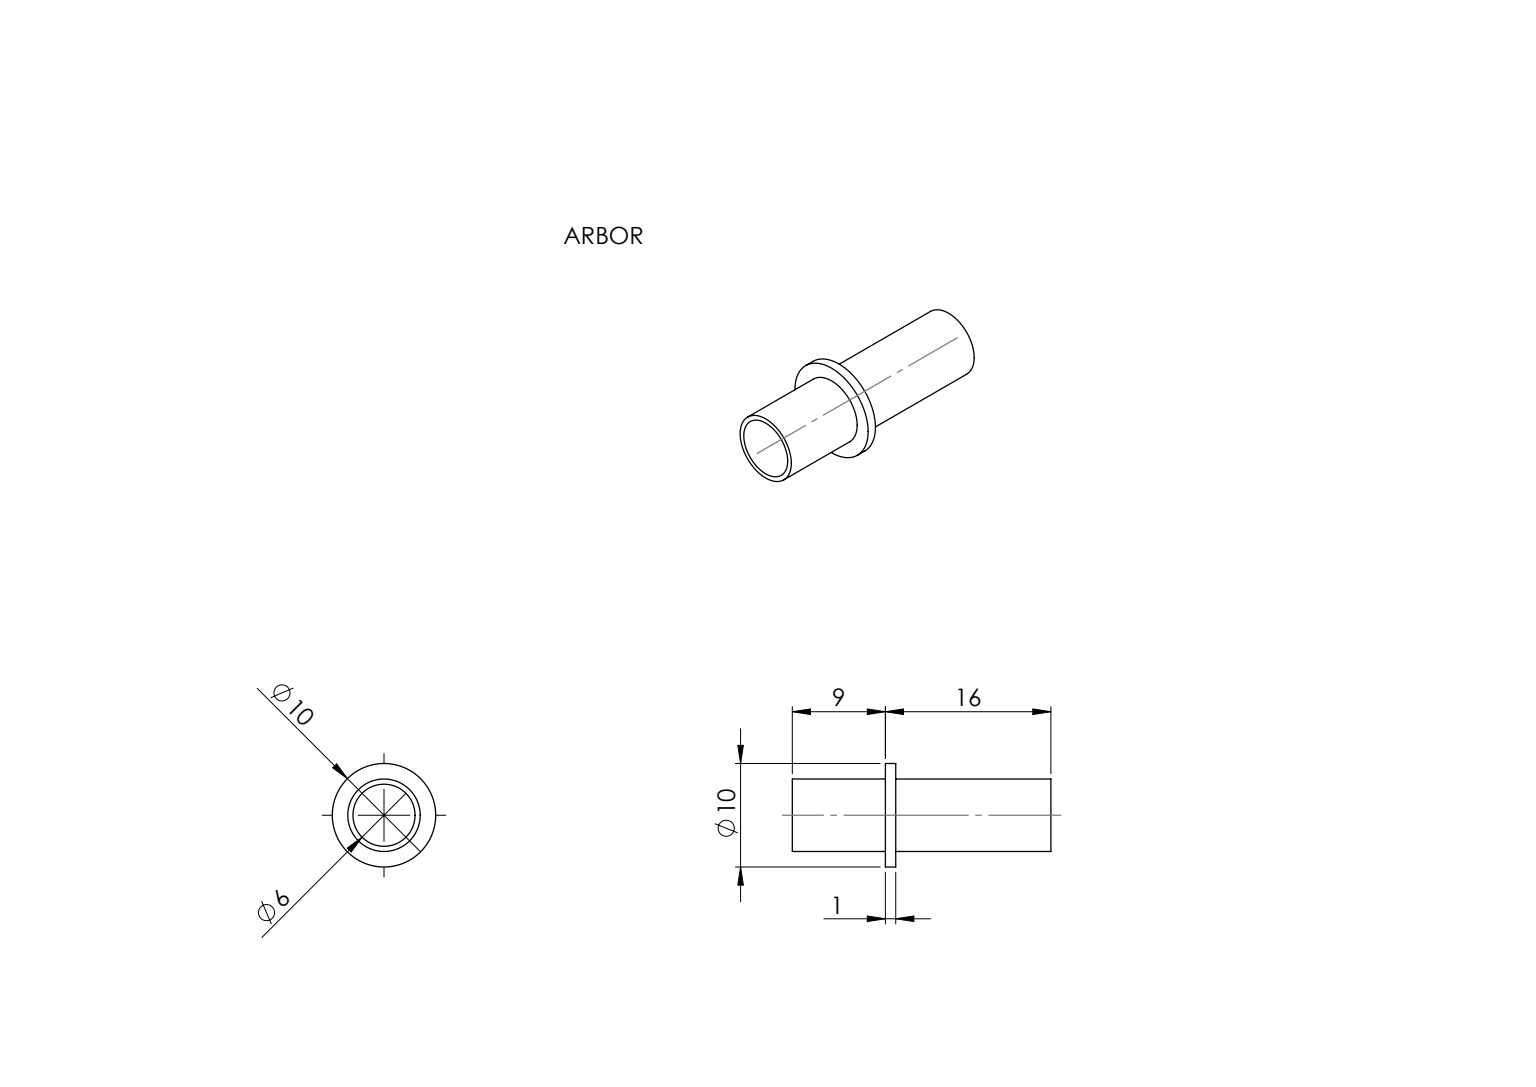
ISO-10303-21;
HEADER;
FILE_DESCRIPTION (('STEP AP214'),
    '1' );
FILE_NAME ('arbor.step',
    '2026-10-08T12:30:53',
    ( '' ),
    ( '' ),
    'SwSTEP 2.0',
    'SolidWorks 2026',
    '' );
FILE_SCHEMA (( 'AUTOMOTIVE_DESIGN' ));
ENDSEC;

DATA;
#87=DIRECTION ( 'NONE',  ( 1.000000000000000000, 0.000000000000000000, 0.000000000000000000 ) ) ;
#239=ORIENTED_EDGE ( 'NONE', *, *, #8409, .T. ) ;
#250=EDGE_LOOP ( 'NONE', ( #5066, #8144, #4716, #4779 ) ) ;
#253=AXIS2_PLACEMENT_3D ( 'NONE', #6645, #1940, #12036 ) ;
#365=EDGE_LOOP ( 'NONE', ( #9600, #8679, #4955, #8031 ) ) ;
#375=DIRECTION ( 'NONE',  ( 0.000000000000000000, 0.000000000000000000, 1.000000000000000000 ) ) ;
#462=EDGE_CURVE ( 'NONE', #4079, #6675, #6924, .T. ) ;
#471=EDGE_LOOP ( 'NONE', ( #5188, #8628, #9006, #4978 ) ) ;
#479=CARTESIAN_POINT ( 'NONE',  ( 0.000000000000000000, 0.000000000000000000, -15.00000000000000000 ) ) ;
#483=MANIFOLD_SOLID_BREP ( 'Boss-Extrude1', #814 ) ;
#506=DIRECTION ( 'NONE',  ( 0.000000000000000000, 0.000000000000000000, 1.000000000000000000 ) ) ;
#541=CARTESIAN_POINT ( 'NONE',  ( 0.000000000000000000, 0.000000000000000000, 1.000000000000000000 ) ) ;
#546=EDGE_LOOP ( 'NONE', ( #8097, #7998 ) ) ;
#571=DIRECTION ( 'NONE',  ( 0.000000000000000000, 0.000000000000000000, 1.000000000000000000 ) ) ;
#619=EDGE_CURVE ( 'NONE', #6675, #1739, #4934, .T. ) ;
#642=LINE ( 'NONE', #3336, #1232 ) ;
#668=FACE_OUTER_BOUND ( 'NONE', #4480, .T. ) ;
#682=EDGE_CURVE ( 'NONE', #9917, #762, #11766, .T. ) ;
#752=( LENGTH_UNIT ( ) NAMED_UNIT ( * ) SI_UNIT ( .MILLI., .METRE. ) );
#762=VERTEX_POINT ( 'NONE', #5708 ) ;
#781=FACE_OUTER_BOUND ( 'NONE', #365, .T. ) ;
#783=DIRECTION ( 'NONE',  ( -0.000000000000000000, -0.000000000000000000, -1.000000000000000000 ) ) ;
#814=CLOSED_SHELL ( 'NONE', ( #10354, #9816, #7402, #7243, #7988, #5762, #1031, #7711, #7647, #5316, #9141, #9675 ) ) ;
#820=DIRECTION ( 'NONE',  ( 1.000000000000000000, 0.000000000000000000, 0.000000000000000000 ) ) ;
#843=VERTEX_POINT ( 'NONE', #1693 ) ;
#927=SURFACE_SIDE_STYLE ('',( #10231 ) ) ;
#967=FACE_BOUND ( 'NONE', #8620, .T. ) ;
#972=AXIS2_PLACEMENT_3D ( 'NONE', #7512, #3791, #8558 ) ;
#1020=CARTESIAN_POINT ( 'NONE',  ( 0.000000000000000000, 0.000000000000000000, 0.000000000000000000 ) ) ;
#1031=ADVANCED_FACE ( 'NONE', ( #3715, #5556 ), #2860, .F. ) ;
#1041=CIRCLE ( 'NONE', #3776, 5.000000000000000000 ) ;
#1061=EDGE_CURVE ( 'NONE', #1959, #9571, #11360, .T. ) ;
#1065=( LENGTH_UNIT ( ) NAMED_UNIT ( * ) SI_UNIT ( .MILLI., .METRE. ) );
#1078=CARTESIAN_POINT ( 'NONE',  ( 0.000000000000000000, 0.000000000000000000, 0.000000000000000000 ) ) ;
#1088=FACE_OUTER_BOUND ( 'NONE', #9309, .T. ) ;
#1202=AXIS2_PLACEMENT_3D ( 'NONE', #1748, #5741, #6528 ) ;
#1232=VECTOR ( 'NONE', #6392, 1000.000000000000000 ) ;
#1264=CARTESIAN_POINT ( 'NONE',  ( 0.000000000000000000, 0.000000000000000000, 0.000000000000000000 ) ) ;
#1298=CYLINDRICAL_SURFACE ( 'NONE', #1709, 3.000000000000000000 ) ;
#1299=CARTESIAN_POINT ( 'NONE',  ( 0.000000000000000000, 0.000000000000000000, 10.00000000000000000 ) ) ;
#1301=EDGE_CURVE ( 'NONE', #3060, #5151, #1371, .T. ) ;
#1326=ADVANCED_BREP_SHAPE_REPRESENTATION ( '', ( #483, #8474 ), #1578 ) ;
#1371=CIRCLE ( 'NONE', #6829, 5.000000000000000000 ) ;
#1374=DIRECTION ( 'NONE',  ( 1.000000000000000000, 0.000000000000000000, 0.000000000000000000 ) ) ;
#1389=EDGE_CURVE ( 'NONE', #843, #3060, #7055, .T. ) ;
#1433=DIRECTION ( 'NONE',  ( 1.000000000000000000, 0.000000000000000000, 0.000000000000000000 ) ) ;
#1476=CIRCLE ( 'NONE', #5971, 3.500000000000000000 ) ;
#1493=DIRECTION ( 'NONE',  ( 1.000000000000000000, 0.000000000000000000, -0.000000000000000000 ) ) ;
#1551=DIRECTION ( 'NONE',  ( 0.000000000000000000, 0.000000000000000000, 1.000000000000000000 ) ) ;
#1578=( GEOMETRIC_REPRESENTATION_CONTEXT ( 3 ) GLOBAL_UNCERTAINTY_ASSIGNED_CONTEXT ( ( #2564 ) ) GLOBAL_UNIT_ASSIGNED_CONTEXT ( ( #752, #2712, #4616 ) ) REPRESENTATION_CONTEXT ( 'NONE', 'WORKASPACE' ) );
#1584=PRODUCT_DEFINITION_CONTEXT ( 'detailed design', #11146, 'design' ) ;
#1609=DIRECTION ( 'NONE',  ( 0.000000000000000000, 0.000000000000000000, 1.000000000000000000 ) ) ;
#1671=VECTOR ( 'NONE', #2711, 1000.000000000000000 ) ;
#1674=CARTESIAN_POINT ( 'NONE',  ( 0.000000000000000000, 0.000000000000000000, 0.000000000000000000 ) ) ;
#1693=CARTESIAN_POINT ( 'NONE',  ( -5.000000000000000000, 0.000000000000000000, 1.000000000000000000 ) ) ;
#1706=VERTEX_POINT ( 'NONE', #3088 ) ;
#1709=AXIS2_PLACEMENT_3D ( 'NONE', #8770, #375, #10664 ) ;
#1739=VERTEX_POINT ( 'NONE', #9689 ) ;
#1744=CARTESIAN_POINT ( 'NONE',  ( 0.000000000000000000, 0.000000000000000000, -15.00000000000000000 ) ) ;
#1748=CARTESIAN_POINT ( 'NONE',  ( 0.000000000000000000, 0.000000000000000000, -15.00000000000000000 ) ) ;
#1757=DIRECTION ( 'NONE',  ( -0.000000000000000000, -0.000000000000000000, -1.000000000000000000 ) ) ;
#1761=CARTESIAN_POINT ( 'NONE',  ( 5.000000000000000000, 6.123233995736766282E-16, 1.000000000000000000 ) ) ;
#1769=CARTESIAN_POINT ( 'NONE',  ( -3.500000000000000000, 4.286263797015736595E-16, 1.000000000000000888 ) ) ;
#1789=ORIENTED_EDGE ( 'NONE', *, *, #6258, .T. ) ;
#1857=CARTESIAN_POINT ( 'NONE',  ( 3.500000000000000000, 0.000000000000000000, 10.00000000000000000 ) ) ;
#1898=ORIENTED_EDGE ( 'NONE', *, *, #7307, .F. ) ;
#1940=DIRECTION ( 'NONE',  ( 0.000000000000000000, 0.000000000000000000, 1.000000000000000000 ) ) ;
#1959=VERTEX_POINT ( 'NONE', #4476 ) ;
#1975=SURFACE_SIDE_STYLE ('',( #9262 ) ) ;
#2010=VECTOR ( 'NONE', #9725, 1000.000000000000000 ) ;
#2019=AXIS2_PLACEMENT_3D ( 'NONE', #541, #783, #6240 ) ;
#2050=AXIS2_PLACEMENT_3D ( 'NONE', #10605, #10721, #2398 ) ;
#2086=DIRECTION ( 'NONE',  ( 1.000000000000000000, 0.000000000000000000, 0.000000000000000000 ) ) ;
#2126=LINE ( 'NONE', #10576, #12103 ) ;
#2185=PRODUCT ( 'arbor', 'arbor', '', ( #4393 ) ) ;
#2315=CARTESIAN_POINT ( 'NONE',  ( -3.500000000000000000, 4.286263797015736595E-16, -15.00000000000000000 ) ) ;
#2336=CARTESIAN_POINT ( 'NONE',  ( 0.000000000000000000, 0.000000000000000000, 1.000000000000000000 ) ) ;
#2349=CARTESIAN_POINT ( 'NONE',  ( 0.000000000000000000, 0.000000000000000000, 1.000000000000000000 ) ) ;
#2398=DIRECTION ( 'NONE',  ( 1.000000000000000000, 0.000000000000000000, 0.000000000000000000 ) ) ;
#2408=CARTESIAN_POINT ( 'NONE',  ( 0.000000000000000000, 0.000000000000000000, 0.000000000000000000 ) ) ;
#2428=CIRCLE ( 'NONE', #2050, 3.000000000000000000 ) ;
#2500=ORIENTED_EDGE ( 'NONE', *, *, #10665, .T. ) ;
#2564=UNCERTAINTY_MEASURE_WITH_UNIT (LENGTH_MEASURE( 1.000000000000000082E-05 ), #752, 'distance_accuracy_value', 'NONE');
#2591=( LENGTH_UNIT ( ) NAMED_UNIT ( * ) SI_UNIT ( .MILLI., .METRE. ) );
#2626=DIRECTION ( 'NONE',  ( 0.000000000000000000, 0.000000000000000000, 1.000000000000000000 ) ) ;
#2653=DIRECTION ( 'NONE',  ( 1.000000000000000000, 0.000000000000000000, 0.000000000000000000 ) ) ;
#2711=DIRECTION ( 'NONE',  ( 0.000000000000000000, 0.000000000000000000, 1.000000000000000000 ) ) ;
#2712=( NAMED_UNIT ( * ) PLANE_ANGLE_UNIT ( ) SI_UNIT ( $, .RADIAN. ) );
#2725=EDGE_CURVE ( 'NONE', #1706, #6294, #2126, .T. ) ;
#2769=ORIENTED_EDGE ( 'NONE', *, *, #8606, .T. ) ;
#2772=ORIENTED_EDGE ( 'NONE', *, *, #6213, .T. ) ;
#2779=CARTESIAN_POINT ( 'NONE',  ( 0.000000000000000000, 0.000000000000000000, 10.00000000000000000 ) ) ;
#2806=EDGE_LOOP ( 'NONE', ( #5585, #10926 ) ) ;
#2812=FACE_OUTER_BOUND ( 'NONE', #7133, .T. ) ;
#2860=PLANE ( 'NONE',  #1202 ) ;
#2862=EDGE_LOOP ( 'NONE', ( #6778, #7942 ) ) ;
#2866=FACE_OUTER_BOUND ( 'NONE', #7146, .T. ) ;
#2875=DIRECTION ( 'NONE',  ( 0.000000000000000000, 0.000000000000000000, 1.000000000000000000 ) ) ;
#2891=AXIS2_PLACEMENT_3D ( 'NONE', #4371, #11831, #7229 ) ;
#2907=CARTESIAN_POINT ( 'NONE',  ( -5.000000000000000000, 0.000000000000000000, 0.000000000000000000 ) ) ;
#2921=ORIENTED_EDGE ( 'NONE', *, *, #12072, .T. ) ;
#2924=CARTESIAN_POINT ( 'NONE',  ( 0.000000000000000000, 0.000000000000000000, -15.00000000000000000 ) ) ;
#3052=DIRECTION ( 'NONE',  ( 1.000000000000000000, 0.000000000000000000, 0.000000000000000000 ) ) ;
#3060=VERTEX_POINT ( 'NONE', #2907 ) ;
#3088=CARTESIAN_POINT ( 'NONE',  ( 3.500000000000000000, 0.000000000000000000, -15.00000000000000000 ) ) ;
#3122=DIRECTION ( 'NONE',  ( 1.000000000000000000, 0.000000000000000000, 0.000000000000000000 ) ) ;
#3146=( GEOMETRIC_REPRESENTATION_CONTEXT ( 3 ) GLOBAL_UNCERTAINTY_ASSIGNED_CONTEXT ( ( #10648 ) ) GLOBAL_UNIT_ASSIGNED_CONTEXT ( ( #1065, #10240, #5651 ) ) REPRESENTATION_CONTEXT ( 'NONE', 'WORKASPACE' ) );
#3159=PRESENTATION_STYLE_ASSIGNMENT (( #8338 ) ) ;
#3171=PRODUCT_DEFINITION_SHAPE ( 'NONE', 'NONE',  #9054 ) ;
#3172=DIRECTION ( 'NONE',  ( 0.000000000000000000, 0.000000000000000000, 1.000000000000000000 ) ) ;
#3259=AXIS2_PLACEMENT_3D ( 'NONE', #4456, #2626, #7318 ) ;
#3276=ORIENTED_EDGE ( 'NONE', *, *, #5053, .F. ) ;
#3315=DIRECTION ( 'NONE',  ( 0.000000000000000000, 0.000000000000000000, 1.000000000000000000 ) ) ;
#3336=CARTESIAN_POINT ( 'NONE',  ( -3.500000000000000000, 4.286263797015736595E-16, -15.00000000000000000 ) ) ;
#3341=ORIENTED_EDGE ( 'NONE', *, *, #682, .F. ) ;
#3392=ORIENTED_EDGE ( 'NONE', *, *, #10688, .F. ) ;
#3650=CYLINDRICAL_SURFACE ( 'NONE', #9938, 3.500000000000000000 ) ;
#3656=DIRECTION ( 'NONE',  ( 1.000000000000000000, 0.000000000000000000, 0.000000000000000000 ) ) ;
#3715=FACE_BOUND ( 'NONE', #2862, .T. ) ;
#3776=AXIS2_PLACEMENT_3D ( 'NONE', #6403, #11185, #10131 ) ;
#3791=DIRECTION ( 'NONE',  ( 0.000000000000000000, 0.000000000000000000, 1.000000000000000000 ) ) ;
#3792=CARTESIAN_POINT ( 'NONE',  ( 0.000000000000000000, 0.000000000000000000, 10.00000000000000000 ) ) ;
#3842=AXIS2_PLACEMENT_3D ( 'NONE', #479, #7763, #7827 ) ;
#3902=ORIENTED_EDGE ( 'NONE', *, *, #619, .T. ) ;
#3922=PRODUCT_DEFINITION_FORMATION_WITH_SPECIFIED_SOURCE ( 'ANY', '', #2185, .NOT_KNOWN. ) ;
#3976=VERTEX_POINT ( 'NONE', #1769 ) ;
#4079=VERTEX_POINT ( 'NONE', #9242 ) ;
#4084=FACE_OUTER_BOUND ( 'NONE', #471, .T. ) ;
#4179=FACE_OUTER_BOUND ( 'NONE', #11279, .T. ) ;
#4183=FILL_AREA_STYLE_COLOUR ( '', #11182 ) ;
#4209=EDGE_LOOP ( 'NONE', ( #7969, #2500 ) ) ;
#4267=SHAPE_DEFINITION_REPRESENTATION ( #3171, #6698 ) ;
#4371=CARTESIAN_POINT ( 'NONE',  ( 0.000000000000000000, 0.000000000000000000, -15.00000000000000000 ) ) ;
#4393=PRODUCT_CONTEXT ( 'NONE', #9663, 'mechanical' ) ;
#4450=ORIENTED_EDGE ( 'NONE', *, *, #10688, .T. ) ;
#4456=CARTESIAN_POINT ( 'NONE',  ( 0.000000000000000000, 0.000000000000000000, -15.00000000000000000 ) ) ;
#4476=CARTESIAN_POINT ( 'NONE',  ( -3.000000000000000000, 3.673940397442059868E-16, -15.00000000000000000 ) ) ;
#4480=EDGE_LOOP ( 'NONE', ( #3392, #239, #2921, #6217 ) ) ;
#4490=DIRECTION ( 'NONE',  ( 0.000000000000000000, 0.000000000000000000, 1.000000000000000000 ) ) ;
#4604=EDGE_CURVE ( 'NONE', #3976, #1739, #642, .T. ) ;
#4616=( NAMED_UNIT ( * ) SI_UNIT ( $, .STERADIAN. ) SOLID_ANGLE_UNIT ( ) );
#4631=DIRECTION ( 'NONE',  ( 0.000000000000000000, 0.000000000000000000, 1.000000000000000000 ) ) ;
#4716=ORIENTED_EDGE ( 'NONE', *, *, #682, .T. ) ;
#4740=CARTESIAN_POINT ( 'NONE',  ( 3.000000000000000000, 0.000000000000000000, -15.00000000000000000 ) ) ;
#4779=ORIENTED_EDGE ( 'NONE', *, *, #10108, .F. ) ;
#4783=AXIS2_PLACEMENT_3D ( 'NONE', #1299, #3315, #7786 ) ;
#4795=SHAPE_REPRESENTATION_RELATIONSHIP ( 'NONE' , 'NONE' ,  #6698, #1326 ) ;
#4809=DIRECTION ( 'NONE',  ( 0.000000000000000000, 0.000000000000000000, 1.000000000000000000 ) ) ;
#4840=CARTESIAN_POINT ( 'NONE',  ( 0.000000000000000000, 0.000000000000000000, 10.00000000000000000 ) ) ;
#4849=SURFACE_STYLE_USAGE ( .BOTH. , #1975 ) ;
#4878=AXIS2_PLACEMENT_3D ( 'NONE', #12037, #10267, #8373 ) ;
#4905=DIRECTION ( 'NONE',  ( 1.000000000000000000, 0.000000000000000000, 0.000000000000000000 ) ) ;
#4934=CIRCLE ( 'NONE', #9624, 3.500000000000000000 ) ;
#4955=ORIENTED_EDGE ( 'NONE', *, *, #619, .F. ) ;
#4978=ORIENTED_EDGE ( 'NONE', *, *, #11157, .T. ) ;
#5044=AXIS2_PLACEMENT_3D ( 'NONE', #2336, #6138, #8657 ) ;
#5053=EDGE_CURVE ( 'NONE', #5601, #10654, #5195, .T. ) ;
#5061=AXIS2_PLACEMENT_3D ( 'NONE', #1078, #4809, #1493 ) ;
#5066=ORIENTED_EDGE ( 'NONE', *, *, #1061, .F. ) ;
#5151=VERTEX_POINT ( 'NONE', #6178 ) ;
#5188=ORIENTED_EDGE ( 'NONE', *, *, #6513, .F. ) ;
#5195=LINE ( 'NONE', #2315, #8077 ) ;
#5267=CIRCLE ( 'NONE', #972, 5.000000000000000000 ) ;
#5316=ADVANCED_FACE ( 'NONE', ( #1088, #11307 ), #10446, .T. ) ;
#5435=CYLINDRICAL_SURFACE ( 'NONE', #2019, 5.000000000000000000 ) ;
#5473=EDGE_LOOP ( 'NONE', ( #3276, #10899, #10857, #10611 ) ) ;
#5483=STYLED_ITEM ( 'NONE', ( #6622 ), #1326 ) ;
#5495=CYLINDRICAL_SURFACE ( 'NONE', #10815, 3.500000000000000000 ) ;
#5500=UNCERTAINTY_MEASURE_WITH_UNIT (LENGTH_MEASURE( 1.000000000000000082E-05 ), #2591, 'distance_accuracy_value', 'NONE');
#5556=FACE_OUTER_BOUND ( 'NONE', #546, .T. ) ;
#5582=( NAMED_UNIT ( * ) PLANE_ANGLE_UNIT ( ) SI_UNIT ( $, .RADIAN. ) );
#5585=ORIENTED_EDGE ( 'NONE', *, *, #1301, .F. ) ;
#5601=VERTEX_POINT ( 'NONE', #7749 ) ;
#5651=( NAMED_UNIT ( * ) SI_UNIT ( $, .STERADIAN. ) SOLID_ANGLE_UNIT ( ) );
#5708=CARTESIAN_POINT ( 'NONE',  ( 3.000000000000000000, 0.000000000000000000, 10.00000000000000000 ) ) ;
#5736=FACE_BOUND ( 'NONE', #11005, .T. ) ;
#5741=DIRECTION ( 'NONE',  ( 0.000000000000000000, 0.000000000000000000, 1.000000000000000000 ) ) ;
#5762=ADVANCED_FACE ( 'NONE', ( #2866 ), #5495, .T. ) ;
#5778=EDGE_CURVE ( 'NONE', #1706, #5601, #9835, .T. ) ;
#5835=AXIS2_PLACEMENT_3D ( 'NONE', #7878, #3172, #3052 ) ;
#5903=MECHANICAL_DESIGN_GEOMETRIC_PRESENTATION_REPRESENTATION('',(#6101),#8652);
#5913=AXIS2_PLACEMENT_3D ( 'NONE', #4840, #8643, #2086 ) ;
#5971=AXIS2_PLACEMENT_3D ( 'NONE', #2408, #506, #1433 ) ;
#5990=ORIENTED_EDGE ( 'NONE', *, *, #462, .T. ) ;
#6101=STYLED_ITEM ( 'NONE', ( #3159 ), #483 ) ;
#6138=DIRECTION ( 'NONE',  ( -0.000000000000000000, -0.000000000000000000, -1.000000000000000000 ) ) ;
#6178=CARTESIAN_POINT ( 'NONE',  ( 5.000000000000000000, 6.123233995736766282E-16, 0.000000000000000000 ) ) ;
#6195=CARTESIAN_POINT ( 'NONE',  ( -3.000000000000000000, 3.673940397442059868E-16, 10.00000000000000000 ) ) ;
#6213=EDGE_CURVE ( 'NONE', #6294, #10654, #10155, .T. ) ;
#6217=ORIENTED_EDGE ( 'NONE', *, *, #1389, .F. ) ;
#6240=DIRECTION ( 'NONE',  ( -1.000000000000000000, 0.000000000000000000, 0.000000000000000000 ) ) ;
#6258=EDGE_CURVE ( 'NONE', #10654, #6294, #1476, .T. ) ;
#6294=VERTEX_POINT ( 'NONE', #9750 ) ;
#6392=DIRECTION ( 'NONE',  ( 0.000000000000000000, 0.000000000000000000, 1.000000000000000000 ) ) ;
#6403=CARTESIAN_POINT ( 'NONE',  ( 0.000000000000000000, 0.000000000000000000, 0.000000000000000000 ) ) ;
#6513=EDGE_CURVE ( 'NONE', #1959, #9917, #8217, .T. ) ;
#6524=DIRECTION ( 'NONE',  ( 1.000000000000000000, 0.000000000000000000, 0.000000000000000000 ) ) ;
#6528=DIRECTION ( 'NONE',  ( 1.000000000000000000, 0.000000000000000000, -0.000000000000000000 ) ) ;
#6622=PRESENTATION_STYLE_ASSIGNMENT (( #4849 ) ) ;
#6645=CARTESIAN_POINT ( 'NONE',  ( 0.000000000000000000, 0.000000000000000000, -15.00000000000000000 ) ) ;
#6675=VERTEX_POINT ( 'NONE', #1857 ) ;
#6698=SHAPE_REPRESENTATION ( 'arbor', ( #8474 ), #1578 ) ;
#6778=ORIENTED_EDGE ( 'NONE', *, *, #11223, .T. ) ;
#6782=FACE_OUTER_BOUND ( 'NONE', #7994, .T. ) ;
#6784=LINE ( 'NONE', #10464, #2010 ) ;
#6829=AXIS2_PLACEMENT_3D ( 'NONE', #1264, #8734, #8911 ) ;
#6924=LINE ( 'NONE', #9986, #8248 ) ;
#6959=ORIENTED_EDGE ( 'NONE', *, *, #8606, .F. ) ;
#6964=ORIENTED_EDGE ( 'NONE', *, *, #1389, .T. ) ;
#6993=AXIS2_PLACEMENT_3D ( 'NONE', #3792, #7513, #10326 ) ;
#7034=LINE ( 'NONE', #10783, #11704 ) ;
#7036=CYLINDRICAL_SURFACE ( 'NONE', #5044, 5.000000000000000000 ) ;
#7051=DIRECTION ( 'NONE',  ( -0.000000000000000000, -0.000000000000000000, -1.000000000000000000 ) ) ;
#7055=LINE ( 'NONE', #10808, #8444 ) ;
#7112=DIRECTION ( 'NONE',  ( 1.000000000000000000, 0.000000000000000000, 0.000000000000000000 ) ) ;
#7133=EDGE_LOOP ( 'NONE', ( #3902, #8113 ) ) ;
#7146=EDGE_LOOP ( 'NONE', ( #8855, #1898, #5990, #7808 ) ) ;
#7229=DIRECTION ( 'NONE',  ( 1.000000000000000000, 0.000000000000000000, 0.000000000000000000 ) ) ;
#7243=ADVANCED_FACE ( 'NONE', ( #6782 ), #7890, .T. ) ;
#7290=AXIS2_PLACEMENT_3D ( 'NONE', #2349, #571, #1374 ) ;
#7307=EDGE_CURVE ( 'NONE', #4079, #3976, #10880, .T. ) ;
#7318=DIRECTION ( 'NONE',  ( 1.000000000000000000, 0.000000000000000000, 0.000000000000000000 ) ) ;
#7402=ADVANCED_FACE ( 'NONE', ( #781 ), #9110, .T. ) ;
#7481=ORIENTED_EDGE ( 'NONE', *, *, #6213, .F. ) ;
#7512=CARTESIAN_POINT ( 'NONE',  ( 0.000000000000000000, 0.000000000000000000, 1.000000000000000000 ) ) ;
#7513=DIRECTION ( 'NONE',  ( 0.000000000000000000, 0.000000000000000000, 1.000000000000000000 ) ) ;
#7647=ADVANCED_FACE ( 'NONE', ( #2812, #967 ), #8446, .T. ) ;
#7695=CIRCLE ( 'NONE', #11031, 3.500000000000000000 ) ;
#7711=ADVANCED_FACE ( 'NONE', ( #4084 ), #11550, .F. ) ;
#7749=CARTESIAN_POINT ( 'NONE',  ( -3.500000000000000000, 4.286263797015736595E-16, -15.00000000000000000 ) ) ;
#7763=DIRECTION ( 'NONE',  ( 0.000000000000000000, 0.000000000000000000, 1.000000000000000000 ) ) ;
#7773=ORIENTED_EDGE ( 'NONE', *, *, #2725, .F. ) ;
#7786=DIRECTION ( 'NONE',  ( 1.000000000000000000, 0.000000000000000000, 0.000000000000000000 ) ) ;
#7808=ORIENTED_EDGE ( 'NONE', *, *, #10812, .F. ) ;
#7827=DIRECTION ( 'NONE',  ( 1.000000000000000000, 0.000000000000000000, 0.000000000000000000 ) ) ;
#7878=CARTESIAN_POINT ( 'NONE',  ( 0.000000000000000000, 0.000000000000000000, -15.00000000000000000 ) ) ;
#7890=CYLINDRICAL_SURFACE ( 'NONE', #3842, 3.500000000000000000 ) ;
#7910=FILL_AREA_STYLE ('',( #4183 ) ) ;
#7942=ORIENTED_EDGE ( 'NONE', *, *, #1061, .T. ) ;
#7969=ORIENTED_EDGE ( 'NONE', *, *, #7307, .T. ) ;
#7988=ADVANCED_FACE ( 'NONE', ( #8055 ), #3650, .T. ) ;
#7994=EDGE_LOOP ( 'NONE', ( #11706, #10429, #7481, #7773 ) ) ;
#7998=ORIENTED_EDGE ( 'NONE', *, *, #9453, .F. ) ;
#8031=ORIENTED_EDGE ( 'NONE', *, *, #462, .F. ) ;
#8036=AXIS2_PLACEMENT_3D ( 'NONE', #9341, #9222, #11116 ) ;
#8055=FACE_OUTER_BOUND ( 'NONE', #5473, .T. ) ;
#8077=VECTOR ( 'NONE', #8810, 1000.000000000000000 ) ;
#8093=CIRCLE ( 'NONE', #7290, 5.000000000000000000 ) ;
#8097=ORIENTED_EDGE ( 'NONE', *, *, #5778, .F. ) ;
#8113=ORIENTED_EDGE ( 'NONE', *, *, #10812, .T. ) ;
#8144=ORIENTED_EDGE ( 'NONE', *, *, #6513, .T. ) ;
#8217=LINE ( 'NONE', #10175, #1671 ) ;
#8248=VECTOR ( 'NONE', #1609, 1000.000000000000000 ) ;
#8314=DIRECTION ( 'NONE',  ( 0.000000000000000000, 0.000000000000000000, 1.000000000000000000 ) ) ;
#8338=SURFACE_STYLE_USAGE ( .BOTH. , #927 ) ;
#8348=FILL_AREA_STYLE ('',( #10176 ) ) ;
#8373=DIRECTION ( 'NONE',  ( 1.000000000000000000, 0.000000000000000000, -0.000000000000000000 ) ) ;
#8409=EDGE_CURVE ( 'NONE', #10512, #5151, #7034, .T. ) ;
#8444=VECTOR ( 'NONE', #11715, 1000.000000000000000 ) ;
#8446=PLANE ( 'NONE',  #6993 ) ;
#8474=AXIS2_PLACEMENT_3D ( 'NONE', #1674, #1551, #2653 ) ;
#8490=DIRECTION ( 'NONE',  ( 0.000000000000000000, 0.000000000000000000, 1.000000000000000000 ) ) ;
#8536=AXIS2_PLACEMENT_3D ( 'NONE', #8701, #10649, #3122 ) ;
#8558=DIRECTION ( 'NONE',  ( 1.000000000000000000, 0.000000000000000000, 0.000000000000000000 ) ) ;
#8606=EDGE_CURVE ( 'NONE', #843, #10512, #5267, .T. ) ;
#8620=EDGE_LOOP ( 'NONE', ( #11824, #3341 ) ) ;
#8628=ORIENTED_EDGE ( 'NONE', *, *, #11223, .F. ) ;
#8643=DIRECTION ( 'NONE',  ( 0.000000000000000000, 0.000000000000000000, 1.000000000000000000 ) ) ;
#8652=( GEOMETRIC_REPRESENTATION_CONTEXT ( 3 ) GLOBAL_UNCERTAINTY_ASSIGNED_CONTEXT ( ( #5500 ) ) GLOBAL_UNIT_ASSIGNED_CONTEXT ( ( #2591, #5582, #10102 ) ) REPRESENTATION_CONTEXT ( 'NONE', 'WORKASPACE' ) );
#8657=DIRECTION ( 'NONE',  ( -1.000000000000000000, 0.000000000000000000, 0.000000000000000000 ) ) ;
#8679=ORIENTED_EDGE ( 'NONE', *, *, #4604, .T. ) ;
#8701=CARTESIAN_POINT ( 'NONE',  ( 0.000000000000000000, 0.000000000000000000, 1.000000000000000888 ) ) ;
#8734=DIRECTION ( 'NONE',  ( 0.000000000000000000, 0.000000000000000000, 1.000000000000000000 ) ) ;
#8770=CARTESIAN_POINT ( 'NONE',  ( 0.000000000000000000, 0.000000000000000000, -15.00000000000000000 ) ) ;
#8810=DIRECTION ( 'NONE',  ( 0.000000000000000000, 0.000000000000000000, 1.000000000000000000 ) ) ;
#8855=ORIENTED_EDGE ( 'NONE', *, *, #4604, .F. ) ;
#8906=CARTESIAN_POINT ( 'NONE',  ( 0.000000000000000000, 0.000000000000000000, 1.000000000000000888 ) ) ;
#8911=DIRECTION ( 'NONE',  ( 1.000000000000000000, 0.000000000000000000, 0.000000000000000000 ) ) ;
#9006=ORIENTED_EDGE ( 'NONE', *, *, #10108, .T. ) ;
#9054=PRODUCT_DEFINITION ( 'UNKNOWN', '', #3922, #1584 ) ;
#9110=CYLINDRICAL_SURFACE ( 'NONE', #3259, 3.500000000000000000 ) ;
#9141=ADVANCED_FACE ( 'NONE', ( #10311, #5736 ), #9461, .F. ) ;
#9222=DIRECTION ( 'NONE',  ( 0.000000000000000000, 0.000000000000000000, 1.000000000000000000 ) ) ;
#9242=CARTESIAN_POINT ( 'NONE',  ( 3.500000000000000000, 0.000000000000000000, 1.000000000000000888 ) ) ;
#9262=SURFACE_STYLE_FILL_AREA ( #8348 ) ;
#9309=EDGE_LOOP ( 'NONE', ( #2769, #4450 ) ) ;
#9341=CARTESIAN_POINT ( 'NONE',  ( 0.000000000000000000, 0.000000000000000000, -15.00000000000000000 ) ) ;
#9438=ORIENTED_EDGE ( 'NONE', *, *, #1301, .T. ) ;
#9453=EDGE_CURVE ( 'NONE', #5601, #1706, #11866, .T. ) ;
#9461=PLANE ( 'NONE',  #5061 ) ;
#9554=DIRECTION ( 'NONE',  ( 0.000000000000000000, 0.000000000000000000, 1.000000000000000000 ) ) ;
#9571=VERTEX_POINT ( 'NONE', #4740 ) ;
#9592=MECHANICAL_DESIGN_GEOMETRIC_PRESENTATION_REPRESENTATION('',(#5483),#3146);
#9600=ORIENTED_EDGE ( 'NONE', *, *, #10665, .F. ) ;
#9624=AXIS2_PLACEMENT_3D ( 'NONE', #10468, #9554, #4905 ) ;
#9663=APPLICATION_CONTEXT ( 'automotive_design' ) ;
#9675=ADVANCED_FACE ( 'NONE', ( #4179 ), #7036, .T. ) ;
#9684=FACE_OUTER_BOUND ( 'NONE', #250, .T. ) ;
#9689=CARTESIAN_POINT ( 'NONE',  ( -3.500000000000000000, 4.286263797015736595E-16, 10.00000000000000000 ) ) ;
#9725=DIRECTION ( 'NONE',  ( 0.000000000000000000, 0.000000000000000000, 1.000000000000000000 ) ) ;
#9750=CARTESIAN_POINT ( 'NONE',  ( 3.500000000000000000, 0.000000000000000000, 0.000000000000000000 ) ) ;
#9816=ADVANCED_FACE ( 'NONE', ( #9684 ), #1298, .F. ) ;
#9835=CIRCLE ( 'NONE', #253, 3.500000000000000000 ) ;
#9881=CARTESIAN_POINT ( 'NONE',  ( -3.500000000000000000, 4.286263797015736595E-16, 0.000000000000000000 ) ) ;
#9917=VERTEX_POINT ( 'NONE', #6195 ) ;
#9938=AXIS2_PLACEMENT_3D ( 'NONE', #1744, #4631, #6524 ) ;
#9986=CARTESIAN_POINT ( 'NONE',  ( 3.500000000000000000, 0.000000000000000000, -15.00000000000000000 ) ) ;
#10102=( NAMED_UNIT ( * ) SI_UNIT ( $, .STERADIAN. ) SOLID_ANGLE_UNIT ( ) );
#10108=EDGE_CURVE ( 'NONE', #9571, #762, #6784, .T. ) ;
#10131=DIRECTION ( 'NONE',  ( 1.000000000000000000, 0.000000000000000000, 0.000000000000000000 ) ) ;
#10155=CIRCLE ( 'NONE', #11718, 3.500000000000000000 ) ;
#10175=CARTESIAN_POINT ( 'NONE',  ( -3.000000000000000000, 3.673940397442059868E-16, -15.00000000000000000 ) ) ;
#10176=FILL_AREA_STYLE_COLOUR ( '', #10374 ) ;
#10231=SURFACE_STYLE_FILL_AREA ( #7910 ) ;
#10240=( NAMED_UNIT ( * ) PLANE_ANGLE_UNIT ( ) SI_UNIT ( $, .RADIAN. ) );
#10267=DIRECTION ( 'NONE',  ( 0.000000000000000000, 0.000000000000000000, 1.000000000000000000 ) ) ;
#10311=FACE_OUTER_BOUND ( 'NONE', #2806, .T. ) ;
#10326=DIRECTION ( 'NONE',  ( 1.000000000000000000, 0.000000000000000000, -0.000000000000000000 ) ) ;
#10354=ADVANCED_FACE ( 'NONE', ( #668 ), #5435, .T. ) ;
#10374=COLOUR_RGB ( '', 0.66274510, 0.83137255, 0.94901961) ;
#10429=ORIENTED_EDGE ( 'NONE', *, *, #5053, .T. ) ;
#10440=CIRCLE ( 'NONE', #4783, 3.000000000000000000 ) ;
#10446=PLANE ( 'NONE',  #4878 ) ;
#10464=CARTESIAN_POINT ( 'NONE',  ( 3.000000000000000000, 0.000000000000000000, -15.00000000000000000 ) ) ;
#10468=CARTESIAN_POINT ( 'NONE',  ( 0.000000000000000000, 0.000000000000000000, 10.00000000000000000 ) ) ;
#10512=VERTEX_POINT ( 'NONE', #1761 ) ;
#10576=CARTESIAN_POINT ( 'NONE',  ( 3.500000000000000000, 0.000000000000000000, -15.00000000000000000 ) ) ;
#10605=CARTESIAN_POINT ( 'NONE',  ( 0.000000000000000000, 0.000000000000000000, -15.00000000000000000 ) ) ;
#10611=ORIENTED_EDGE ( 'NONE', *, *, #6258, .F. ) ;
#10648=UNCERTAINTY_MEASURE_WITH_UNIT (LENGTH_MEASURE( 1.000000000000000082E-05 ), #1065, 'distance_accuracy_value', 'NONE');
#10649=DIRECTION ( 'NONE',  ( -0.000000000000000000, -0.000000000000000000, -1.000000000000000000 ) ) ;
#10654=VERTEX_POINT ( 'NONE', #9881 ) ;
#10664=DIRECTION ( 'NONE',  ( 1.000000000000000000, 0.000000000000000000, 0.000000000000000000 ) ) ;
#10665=EDGE_CURVE ( 'NONE', #3976, #4079, #11417, .T. ) ;
#10688=EDGE_CURVE ( 'NONE', #10512, #843, #8093, .T. ) ;
#10721=DIRECTION ( 'NONE',  ( 0.000000000000000000, 0.000000000000000000, 1.000000000000000000 ) ) ;
#10783=CARTESIAN_POINT ( 'NONE',  ( 5.000000000000000000, 6.123233995736766282E-16, 1.000000000000000000 ) ) ;
#10808=CARTESIAN_POINT ( 'NONE',  ( -5.000000000000000000, 0.000000000000000000, 1.000000000000000000 ) ) ;
#10812=EDGE_CURVE ( 'NONE', #1739, #6675, #7695, .T. ) ;
#10815=AXIS2_PLACEMENT_3D ( 'NONE', #2924, #8314, #3656 ) ;
#10830=AXIS2_PLACEMENT_3D ( 'NONE', #8906, #7051, #7112 ) ;
#10857=ORIENTED_EDGE ( 'NONE', *, *, #2725, .T. ) ;
#10880=CIRCLE ( 'NONE', #8536, 3.500000000000000000 ) ;
#10899=ORIENTED_EDGE ( 'NONE', *, *, #9453, .T. ) ;
#10926=ORIENTED_EDGE ( 'NONE', *, *, #12072, .F. ) ;
#11005=EDGE_LOOP ( 'NONE', ( #2772, #1789 ) ) ;
#11031=AXIS2_PLACEMENT_3D ( 'NONE', #2779, #4490, #820 ) ;
#11116=DIRECTION ( 'NONE',  ( 1.000000000000000000, 0.000000000000000000, 0.000000000000000000 ) ) ;
#11146=APPLICATION_CONTEXT ( 'automotive_design' ) ;
#11157=EDGE_CURVE ( 'NONE', #762, #9917, #10440, .T. ) ;
#11182=COLOUR_RGB ( '', 0.66274510, 0.83137255, 0.94901961) ;
#11185=DIRECTION ( 'NONE',  ( 0.000000000000000000, 0.000000000000000000, 1.000000000000000000 ) ) ;
#11223=EDGE_CURVE ( 'NONE', #9571, #1959, #2428, .T. ) ;
#11279=EDGE_LOOP ( 'NONE', ( #11669, #6959, #6964, #9438 ) ) ;
#11307=FACE_BOUND ( 'NONE', #4209, .T. ) ;
#11360=CIRCLE ( 'NONE', #8036, 3.000000000000000000 ) ;
#11417=CIRCLE ( 'NONE', #10830, 3.500000000000000000 ) ;
#11550=CYLINDRICAL_SURFACE ( 'NONE', #5835, 3.000000000000000000 ) ;
#11669=ORIENTED_EDGE ( 'NONE', *, *, #8409, .F. ) ;
#11704=VECTOR ( 'NONE', #1757, 1000.000000000000000 ) ;
#11706=ORIENTED_EDGE ( 'NONE', *, *, #5778, .T. ) ;
#11715=DIRECTION ( 'NONE',  ( -0.000000000000000000, -0.000000000000000000, -1.000000000000000000 ) ) ;
#11718=AXIS2_PLACEMENT_3D ( 'NONE', #1020, #8490, #87 ) ;
#11766=CIRCLE ( 'NONE', #5913, 3.000000000000000000 ) ;
#11824=ORIENTED_EDGE ( 'NONE', *, *, #11157, .F. ) ;
#11831=DIRECTION ( 'NONE',  ( 0.000000000000000000, 0.000000000000000000, 1.000000000000000000 ) ) ;
#11866=CIRCLE ( 'NONE', #2891, 3.500000000000000000 ) ;
#12036=DIRECTION ( 'NONE',  ( 1.000000000000000000, 0.000000000000000000, 0.000000000000000000 ) ) ;
#12037=CARTESIAN_POINT ( 'NONE',  ( 0.000000000000000000, 0.000000000000000000, 1.000000000000000000 ) ) ;
#12072=EDGE_CURVE ( 'NONE', #5151, #3060, #1041, .T. ) ;
#12103=VECTOR ( 'NONE', #2875, 1000.000000000000000 ) ;
ENDSEC;
END-ISO-10303-21;
